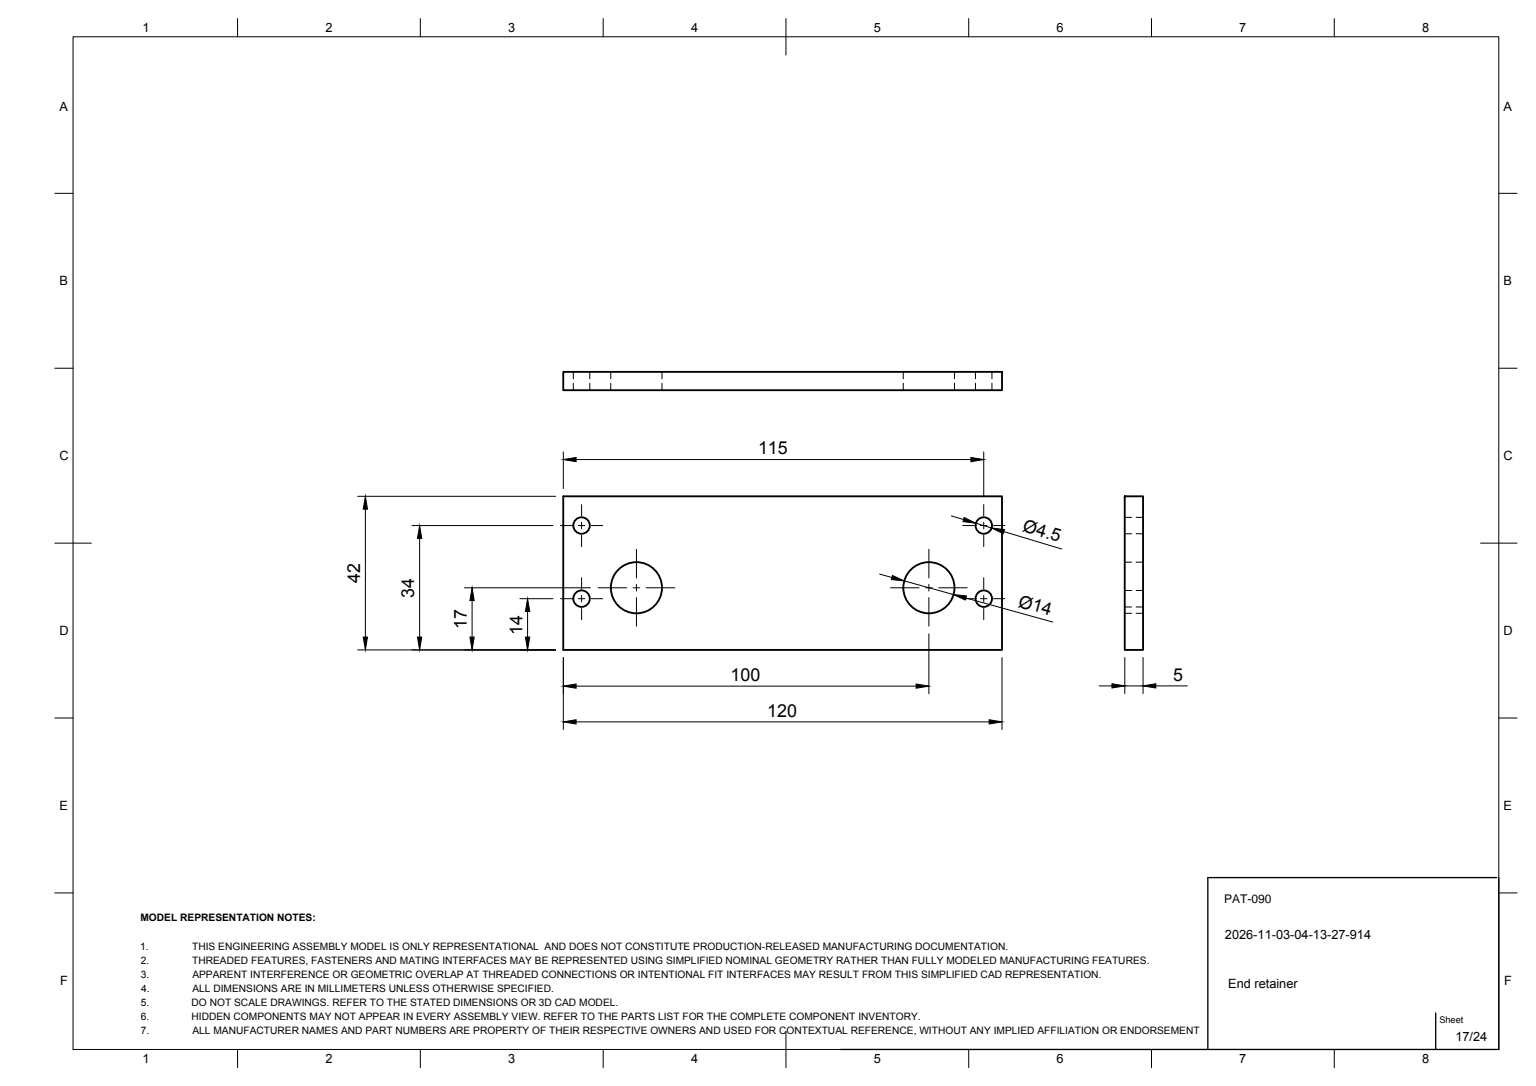
ISO-10303-21;
HEADER;
/* Generated by software containing ST-Developer
 * from STEP Tools, Inc. (www.steptools.com) 
 */

FILE_DESCRIPTION(
/* description */ ('Round-Shaft Linear Stage with Ball Bushings'),
/* implementation_level */ '2;1');

FILE_NAME(
/* name */ 'End retainer.step',
/* time_stamp */ '2026-10-27T10:47:55-07:00',
/* author */ (''),
/* organization */ (''),
/* preprocessor_version */ 'ST-DEVELOPER v20.2',
/* originating_system */ 'Autodesk Translation Framework v15.17.0.0',
/* authorisation */ '');

FILE_SCHEMA (('AUTOMOTIVE_DESIGN { 1 0 10303 214 3 1 1 }'));
ENDSEC;

DATA;
#10=MECHANICAL_DESIGN_GEOMETRIC_PRESENTATION_REPRESENTATION('',(#313),#7835);
#271=SHAPE_REPRESENTATION_RELATIONSHIP('SRR','None',#7960,#292);
#292=ADVANCED_BREP_SHAPE_REPRESENTATION('',(#333),#7824);
#313=STYLED_ITEM('',(#8130),#333);
#333=MANIFOLD_SOLID_BREP('Body1',#4404);
#407=FACE_BOUND('',#1086,.T.);
#408=FACE_BOUND('',#1087,.T.);
#409=FACE_BOUND('',#1088,.T.);
#410=FACE_BOUND('',#1089,.T.);
#411=FACE_BOUND('',#1090,.T.);
#412=FACE_BOUND('',#1091,.T.);
#413=FACE_BOUND('',#1094,.T.);
#414=FACE_BOUND('',#1095,.T.);
#415=FACE_BOUND('',#1096,.T.);
#416=FACE_BOUND('',#1097,.T.);
#417=FACE_BOUND('',#1098,.T.);
#418=FACE_BOUND('',#1099,.T.);
#544=PLANE('',#4921);
#545=PLANE('',#4922);
#546=PLANE('',#4923);
#547=PLANE('',#4924);
#548=PLANE('',#4925);
#549=PLANE('',#4926);
#754=FACE_OUTER_BOUND('',#1078,.T.);
#755=FACE_OUTER_BOUND('',#1079,.T.);
#756=FACE_OUTER_BOUND('',#1080,.T.);
#757=FACE_OUTER_BOUND('',#1081,.T.);
#758=FACE_OUTER_BOUND('',#1082,.T.);
#759=FACE_OUTER_BOUND('',#1083,.T.);
#760=FACE_OUTER_BOUND('',#1084,.T.);
#761=FACE_OUTER_BOUND('',#1085,.T.);
#762=FACE_OUTER_BOUND('',#1092,.T.);
#763=FACE_OUTER_BOUND('',#1093,.T.);
#764=FACE_OUTER_BOUND('',#1100,.T.);
#765=FACE_OUTER_BOUND('',#1101,.T.);
#1078=EDGE_LOOP('',(#3566,#3567,#3568,#3569));
#1079=EDGE_LOOP('',(#3570,#3571,#3572,#3573));
#1080=EDGE_LOOP('',(#3574,#3575,#3576,#3577));
#1081=EDGE_LOOP('',(#3578,#3579,#3580,#3581));
#1082=EDGE_LOOP('',(#3582,#3583,#3584,#3585));
#1083=EDGE_LOOP('',(#3586,#3587,#3588,#3589));
#1084=EDGE_LOOP('',(#3590,#3591,#3592,#3593));
#1085=EDGE_LOOP('',(#3594,#3595,#3596,#3597));
#1086=EDGE_LOOP('',(#3598));
#1087=EDGE_LOOP('',(#3599));
#1088=EDGE_LOOP('',(#3600));
#1089=EDGE_LOOP('',(#3601));
#1090=EDGE_LOOP('',(#3602));
#1091=EDGE_LOOP('',(#3603));
#1092=EDGE_LOOP('',(#3604,#3605,#3606,#3607));
#1093=EDGE_LOOP('',(#3608,#3609,#3610,#3611));
#1094=EDGE_LOOP('',(#3612));
#1095=EDGE_LOOP('',(#3613));
#1096=EDGE_LOOP('',(#3614));
#1097=EDGE_LOOP('',(#3615));
#1098=EDGE_LOOP('',(#3616));
#1099=EDGE_LOOP('',(#3617));
#1100=EDGE_LOOP('',(#3618,#3619,#3620,#3621));
#1101=EDGE_LOOP('',(#3622,#3623,#3624,#3625));
#1434=LINE('',#7202,#1774);
#1435=LINE('',#7208,#1775);
#1436=LINE('',#7214,#1776);
#1437=LINE('',#7220,#1777);
#1438=LINE('',#7226,#1778);
#1439=LINE('',#7232,#1779);
#1440=LINE('',#7237,#1780);
#1441=LINE('',#7239,#1781);
#1442=LINE('',#7241,#1782);
#1443=LINE('',#7242,#1783);
#1444=LINE('',#7245,#1784);
#1445=LINE('',#7247,#1785);
#1446=LINE('',#7248,#1786);
#1447=LINE('',#7251,#1787);
#1448=LINE('',#7253,#1788);
#1449=LINE('',#7254,#1789);
#1450=LINE('',#7256,#1790);
#1451=LINE('',#7257,#1791);
#1774=VECTOR('',#5873,0.225);
#1775=VECTOR('',#5880,0.225);
#1776=VECTOR('',#5887,0.225);
#1777=VECTOR('',#5894,0.225);
#1778=VECTOR('',#5901,0.7);
#1779=VECTOR('',#5908,0.7);
#1780=VECTOR('',#5913,1.);
#1781=VECTOR('',#5914,1.);
#1782=VECTOR('',#5915,1.);
#1783=VECTOR('',#5916,1.);
#1784=VECTOR('',#5919,1.);
#1785=VECTOR('',#5920,1.);
#1786=VECTOR('',#5921,1.);
#1787=VECTOR('',#5924,1.);
#1788=VECTOR('',#5925,1.);
#1789=VECTOR('',#5926,1.);
#1790=VECTOR('',#5929,1.);
#1791=VECTOR('',#5930,1.);
#2030=CIRCLE('',#4904,0.225);
#2031=CIRCLE('',#4905,0.225);
#2032=CIRCLE('',#4907,0.225);
#2033=CIRCLE('',#4908,0.225);
#2034=CIRCLE('',#4910,0.225);
#2035=CIRCLE('',#4911,0.225);
#2036=CIRCLE('',#4913,0.225);
#2037=CIRCLE('',#4914,0.225);
#2038=CIRCLE('',#4916,0.7);
#2039=CIRCLE('',#4917,0.7);
#2040=CIRCLE('',#4919,0.7);
#2041=CIRCLE('',#4920,0.7);
#2307=VERTEX_POINT('',#7199);
#2308=VERTEX_POINT('',#7201);
#2309=VERTEX_POINT('',#7205);
#2310=VERTEX_POINT('',#7207);
#2311=VERTEX_POINT('',#7211);
#2312=VERTEX_POINT('',#7213);
#2313=VERTEX_POINT('',#7217);
#2314=VERTEX_POINT('',#7219);
#2315=VERTEX_POINT('',#7223);
#2316=VERTEX_POINT('',#7225);
#2317=VERTEX_POINT('',#7229);
#2318=VERTEX_POINT('',#7231);
#2319=VERTEX_POINT('',#7235);
#2320=VERTEX_POINT('',#7236);
#2321=VERTEX_POINT('',#7238);
#2322=VERTEX_POINT('',#7240);
#2323=VERTEX_POINT('',#7244);
#2324=VERTEX_POINT('',#7246);
#2325=VERTEX_POINT('',#7250);
#2326=VERTEX_POINT('',#7252);
#2751=EDGE_CURVE('',#2307,#2307,#2030,.T.);
#2752=EDGE_CURVE('',#2307,#2308,#1434,.T.);
#2753=EDGE_CURVE('',#2308,#2308,#2031,.T.);
#2754=EDGE_CURVE('',#2309,#2309,#2032,.T.);
#2755=EDGE_CURVE('',#2309,#2310,#1435,.T.);
#2756=EDGE_CURVE('',#2310,#2310,#2033,.T.);
#2757=EDGE_CURVE('',#2311,#2311,#2034,.T.);
#2758=EDGE_CURVE('',#2311,#2312,#1436,.T.);
#2759=EDGE_CURVE('',#2312,#2312,#2035,.T.);
#2760=EDGE_CURVE('',#2313,#2313,#2036,.T.);
#2761=EDGE_CURVE('',#2313,#2314,#1437,.T.);
#2762=EDGE_CURVE('',#2314,#2314,#2037,.T.);
#2763=EDGE_CURVE('',#2315,#2315,#2038,.T.);
#2764=EDGE_CURVE('',#2315,#2316,#1438,.T.);
#2765=EDGE_CURVE('',#2316,#2316,#2039,.T.);
#2766=EDGE_CURVE('',#2317,#2317,#2040,.T.);
#2767=EDGE_CURVE('',#2317,#2318,#1439,.T.);
#2768=EDGE_CURVE('',#2318,#2318,#2041,.T.);
#2769=EDGE_CURVE('',#2319,#2320,#1440,.T.);
#2770=EDGE_CURVE('',#2320,#2321,#1441,.T.);
#2771=EDGE_CURVE('',#2322,#2321,#1442,.T.);
#2772=EDGE_CURVE('',#2319,#2322,#1443,.T.);
#2773=EDGE_CURVE('',#2323,#2319,#1444,.T.);
#2774=EDGE_CURVE('',#2324,#2322,#1445,.T.);
#2775=EDGE_CURVE('',#2323,#2324,#1446,.T.);
#2776=EDGE_CURVE('',#2325,#2323,#1447,.T.);
#2777=EDGE_CURVE('',#2326,#2324,#1448,.T.);
#2778=EDGE_CURVE('',#2325,#2326,#1449,.T.);
#2779=EDGE_CURVE('',#2320,#2325,#1450,.T.);
#2780=EDGE_CURVE('',#2321,#2326,#1451,.T.);
#3566=ORIENTED_EDGE('',*,*,#2751,.F.);
#3567=ORIENTED_EDGE('',*,*,#2752,.T.);
#3568=ORIENTED_EDGE('',*,*,#2753,.F.);
#3569=ORIENTED_EDGE('',*,*,#2752,.F.);
#3570=ORIENTED_EDGE('',*,*,#2754,.F.);
#3571=ORIENTED_EDGE('',*,*,#2755,.T.);
#3572=ORIENTED_EDGE('',*,*,#2756,.F.);
#3573=ORIENTED_EDGE('',*,*,#2755,.F.);
#3574=ORIENTED_EDGE('',*,*,#2757,.F.);
#3575=ORIENTED_EDGE('',*,*,#2758,.T.);
#3576=ORIENTED_EDGE('',*,*,#2759,.F.);
#3577=ORIENTED_EDGE('',*,*,#2758,.F.);
#3578=ORIENTED_EDGE('',*,*,#2760,.F.);
#3579=ORIENTED_EDGE('',*,*,#2761,.T.);
#3580=ORIENTED_EDGE('',*,*,#2762,.F.);
#3581=ORIENTED_EDGE('',*,*,#2761,.F.);
#3582=ORIENTED_EDGE('',*,*,#2763,.F.);
#3583=ORIENTED_EDGE('',*,*,#2764,.T.);
#3584=ORIENTED_EDGE('',*,*,#2765,.F.);
#3585=ORIENTED_EDGE('',*,*,#2764,.F.);
#3586=ORIENTED_EDGE('',*,*,#2766,.F.);
#3587=ORIENTED_EDGE('',*,*,#2767,.T.);
#3588=ORIENTED_EDGE('',*,*,#2768,.F.);
#3589=ORIENTED_EDGE('',*,*,#2767,.F.);
#3590=ORIENTED_EDGE('',*,*,#2769,.T.);
#3591=ORIENTED_EDGE('',*,*,#2770,.T.);
#3592=ORIENTED_EDGE('',*,*,#2771,.F.);
#3593=ORIENTED_EDGE('',*,*,#2772,.F.);
#3594=ORIENTED_EDGE('',*,*,#2773,.T.);
#3595=ORIENTED_EDGE('',*,*,#2772,.T.);
#3596=ORIENTED_EDGE('',*,*,#2774,.F.);
#3597=ORIENTED_EDGE('',*,*,#2775,.F.);
#3598=ORIENTED_EDGE('',*,*,#2768,.T.);
#3599=ORIENTED_EDGE('',*,*,#2765,.T.);
#3600=ORIENTED_EDGE('',*,*,#2762,.T.);
#3601=ORIENTED_EDGE('',*,*,#2759,.T.);
#3602=ORIENTED_EDGE('',*,*,#2756,.T.);
#3603=ORIENTED_EDGE('',*,*,#2753,.T.);
#3604=ORIENTED_EDGE('',*,*,#2776,.T.);
#3605=ORIENTED_EDGE('',*,*,#2775,.T.);
#3606=ORIENTED_EDGE('',*,*,#2777,.F.);
#3607=ORIENTED_EDGE('',*,*,#2778,.F.);
#3608=ORIENTED_EDGE('',*,*,#2779,.T.);
#3609=ORIENTED_EDGE('',*,*,#2778,.T.);
#3610=ORIENTED_EDGE('',*,*,#2780,.F.);
#3611=ORIENTED_EDGE('',*,*,#2770,.F.);
#3612=ORIENTED_EDGE('',*,*,#2766,.T.);
#3613=ORIENTED_EDGE('',*,*,#2763,.T.);
#3614=ORIENTED_EDGE('',*,*,#2760,.T.);
#3615=ORIENTED_EDGE('',*,*,#2757,.T.);
#3616=ORIENTED_EDGE('',*,*,#2754,.T.);
#3617=ORIENTED_EDGE('',*,*,#2751,.T.);
#3618=ORIENTED_EDGE('',*,*,#2780,.T.);
#3619=ORIENTED_EDGE('',*,*,#2777,.T.);
#3620=ORIENTED_EDGE('',*,*,#2774,.T.);
#3621=ORIENTED_EDGE('',*,*,#2771,.T.);
#3622=ORIENTED_EDGE('',*,*,#2779,.F.);
#3623=ORIENTED_EDGE('',*,*,#2769,.F.);
#3624=ORIENTED_EDGE('',*,*,#2773,.F.);
#3625=ORIENTED_EDGE('',*,*,#2776,.F.);
#4100=CYLINDRICAL_SURFACE('',#4903,0.225);
#4101=CYLINDRICAL_SURFACE('',#4906,0.225);
#4102=CYLINDRICAL_SURFACE('',#4909,0.225);
#4103=CYLINDRICAL_SURFACE('',#4912,0.225);
#4104=CYLINDRICAL_SURFACE('',#4915,0.7);
#4105=CYLINDRICAL_SURFACE('',#4918,0.7);
#4273=ADVANCED_FACE('',(#754),#4100,.F.);
#4274=ADVANCED_FACE('',(#755),#4101,.F.);
#4275=ADVANCED_FACE('',(#756),#4102,.F.);
#4276=ADVANCED_FACE('',(#757),#4103,.F.);
#4277=ADVANCED_FACE('',(#758),#4104,.F.);
#4278=ADVANCED_FACE('',(#759),#4105,.F.);
#4279=ADVANCED_FACE('',(#760),#544,.T.);
#4280=ADVANCED_FACE('',(#761,#407,#408,#409,#410,#411,#412),#545,.T.);
#4281=ADVANCED_FACE('',(#762),#546,.T.);
#4282=ADVANCED_FACE('',(#763,#413,#414,#415,#416,#417,#418),#547,.T.);
#4283=ADVANCED_FACE('',(#764),#548,.T.);
#4284=ADVANCED_FACE('',(#765),#549,.F.);
#4404=CLOSED_SHELL('',(#4273,#4274,#4275,#4276,#4277,#4278,#4279,#4280,
#4281,#4282,#4283,#4284));
#4902=AXIS2_PLACEMENT_3D('',#7197,#5867,#5868);
#4903=AXIS2_PLACEMENT_3D('',#7198,#5869,#5870);
#4904=AXIS2_PLACEMENT_3D('',#7200,#5871,#5872);
#4905=AXIS2_PLACEMENT_3D('',#7203,#5874,#5875);
#4906=AXIS2_PLACEMENT_3D('',#7204,#5876,#5877);
#4907=AXIS2_PLACEMENT_3D('',#7206,#5878,#5879);
#4908=AXIS2_PLACEMENT_3D('',#7209,#5881,#5882);
#4909=AXIS2_PLACEMENT_3D('',#7210,#5883,#5884);
#4910=AXIS2_PLACEMENT_3D('',#7212,#5885,#5886);
#4911=AXIS2_PLACEMENT_3D('',#7215,#5888,#5889);
#4912=AXIS2_PLACEMENT_3D('',#7216,#5890,#5891);
#4913=AXIS2_PLACEMENT_3D('',#7218,#5892,#5893);
#4914=AXIS2_PLACEMENT_3D('',#7221,#5895,#5896);
#4915=AXIS2_PLACEMENT_3D('',#7222,#5897,#5898);
#4916=AXIS2_PLACEMENT_3D('',#7224,#5899,#5900);
#4917=AXIS2_PLACEMENT_3D('',#7227,#5902,#5903);
#4918=AXIS2_PLACEMENT_3D('',#7228,#5904,#5905);
#4919=AXIS2_PLACEMENT_3D('',#7230,#5906,#5907);
#4920=AXIS2_PLACEMENT_3D('',#7233,#5909,#5910);
#4921=AXIS2_PLACEMENT_3D('',#7234,#5911,#5912);
#4922=AXIS2_PLACEMENT_3D('',#7243,#5917,#5918);
#4923=AXIS2_PLACEMENT_3D('',#7249,#5922,#5923);
#4924=AXIS2_PLACEMENT_3D('',#7255,#5927,#5928);
#4925=AXIS2_PLACEMENT_3D('',#7258,#5931,#5932);
#4926=AXIS2_PLACEMENT_3D('',#7259,#5933,#5934);
#5867=DIRECTION('axis',(0.,0.,1.));
#5868=DIRECTION('refdir',(1.,0.,0.));
#5869=DIRECTION('center_axis',(1.,0.,0.));
#5870=DIRECTION('ref_axis',(0.,0.,-1.));
#5871=DIRECTION('center_axis',(1.,0.,0.));
#5872=DIRECTION('ref_axis',(0.,0.,-1.));
#5873=DIRECTION('',(1.,0.,0.));
#5874=DIRECTION('center_axis',(-1.,0.,0.));
#5875=DIRECTION('ref_axis',(0.,0.,-1.));
#5876=DIRECTION('center_axis',(1.,0.,0.));
#5877=DIRECTION('ref_axis',(0.,0.,-1.));
#5878=DIRECTION('center_axis',(1.,0.,0.));
#5879=DIRECTION('ref_axis',(0.,0.,-1.));
#5880=DIRECTION('',(1.,0.,0.));
#5881=DIRECTION('center_axis',(-1.,0.,0.));
#5882=DIRECTION('ref_axis',(0.,0.,-1.));
#5883=DIRECTION('center_axis',(1.,0.,0.));
#5884=DIRECTION('ref_axis',(0.,0.,-1.));
#5885=DIRECTION('center_axis',(1.,0.,0.));
#5886=DIRECTION('ref_axis',(0.,0.,-1.));
#5887=DIRECTION('',(1.,0.,0.));
#5888=DIRECTION('center_axis',(-1.,0.,0.));
#5889=DIRECTION('ref_axis',(0.,0.,-1.));
#5890=DIRECTION('center_axis',(1.,0.,0.));
#5891=DIRECTION('ref_axis',(0.,0.,-1.));
#5892=DIRECTION('center_axis',(1.,0.,0.));
#5893=DIRECTION('ref_axis',(0.,0.,-1.));
#5894=DIRECTION('',(1.,0.,0.));
#5895=DIRECTION('center_axis',(-1.,0.,0.));
#5896=DIRECTION('ref_axis',(0.,0.,-1.));
#5897=DIRECTION('center_axis',(1.,0.,0.));
#5898=DIRECTION('ref_axis',(0.,0.,-1.));
#5899=DIRECTION('center_axis',(1.,0.,0.));
#5900=DIRECTION('ref_axis',(0.,0.,-1.));
#5901=DIRECTION('',(1.,0.,0.));
#5902=DIRECTION('center_axis',(-1.,0.,0.));
#5903=DIRECTION('ref_axis',(0.,0.,-1.));
#5904=DIRECTION('center_axis',(1.,0.,0.));
#5905=DIRECTION('ref_axis',(0.,0.,-1.));
#5906=DIRECTION('center_axis',(1.,0.,0.));
#5907=DIRECTION('ref_axis',(0.,0.,-1.));
#5908=DIRECTION('',(1.,0.,0.));
#5909=DIRECTION('center_axis',(-1.,0.,0.));
#5910=DIRECTION('ref_axis',(0.,0.,-1.));
#5911=DIRECTION('center_axis',(0.,1.,0.));
#5912=DIRECTION('ref_axis',(-1.,0.,0.));
#5913=DIRECTION('',(-1.,0.,0.));
#5914=DIRECTION('',(0.,0.,1.));
#5915=DIRECTION('',(-1.,0.,0.));
#5916=DIRECTION('',(0.,0.,1.));
#5917=DIRECTION('center_axis',(1.,0.,0.));
#5918=DIRECTION('ref_axis',(0.,1.,0.));
#5919=DIRECTION('',(0.,1.,0.));
#5920=DIRECTION('',(0.,1.,0.));
#5921=DIRECTION('',(0.,0.,1.));
#5922=DIRECTION('center_axis',(0.,-1.,0.));
#5923=DIRECTION('ref_axis',(1.,0.,0.));
#5924=DIRECTION('',(1.,0.,0.));
#5925=DIRECTION('',(1.,0.,0.));
#5926=DIRECTION('',(0.,0.,1.));
#5927=DIRECTION('center_axis',(-1.,0.,0.));
#5928=DIRECTION('ref_axis',(0.,-1.,0.));
#5929=DIRECTION('',(0.,-1.,0.));
#5930=DIRECTION('',(0.,-1.,0.));
#5931=DIRECTION('center_axis',(0.,0.,1.));
#5932=DIRECTION('ref_axis',(1.,0.,0.));
#5933=DIRECTION('center_axis',(0.,0.,1.));
#5934=DIRECTION('ref_axis',(1.,0.,0.));
#7197=CARTESIAN_POINT('',(0.,0.,0.));
#7198=CARTESIAN_POINT('Origin',(9.9,5.5,3.));
#7199=CARTESIAN_POINT('',(10.,5.5,3.225));
#7200=CARTESIAN_POINT('Origin',(10.,5.5,3.));
#7201=CARTESIAN_POINT('',(10.5,5.5,3.225));
#7202=CARTESIAN_POINT('',(9.9,5.5,3.225));
#7203=CARTESIAN_POINT('Origin',(10.5,5.5,3.));
#7204=CARTESIAN_POINT('Origin',(9.9,-5.5,5.));
#7205=CARTESIAN_POINT('',(10.,-5.5,5.225));
#7206=CARTESIAN_POINT('Origin',(10.,-5.5,5.));
#7207=CARTESIAN_POINT('',(10.5,-5.5,5.225));
#7208=CARTESIAN_POINT('',(9.9,-5.5,5.225));
#7209=CARTESIAN_POINT('Origin',(10.5,-5.5,5.));
#7210=CARTESIAN_POINT('Origin',(9.9,-5.5,3.));
#7211=CARTESIAN_POINT('',(10.,-5.5,3.225));
#7212=CARTESIAN_POINT('Origin',(10.,-5.5,3.));
#7213=CARTESIAN_POINT('',(10.5,-5.5,3.225));
#7214=CARTESIAN_POINT('',(9.9,-5.5,3.225));
#7215=CARTESIAN_POINT('Origin',(10.5,-5.5,3.));
#7216=CARTESIAN_POINT('Origin',(9.9,5.5,5.));
#7217=CARTESIAN_POINT('',(10.,5.5,5.225));
#7218=CARTESIAN_POINT('Origin',(10.,5.5,5.));
#7219=CARTESIAN_POINT('',(10.5,5.5,5.225));
#7220=CARTESIAN_POINT('',(9.9,5.5,5.225));
#7221=CARTESIAN_POINT('Origin',(10.5,5.5,5.));
#7222=CARTESIAN_POINT('Origin',(9.9,-4.,3.3));
#7223=CARTESIAN_POINT('',(10.,-4.,4.));
#7224=CARTESIAN_POINT('Origin',(10.,-4.,3.3));
#7225=CARTESIAN_POINT('',(10.5,-4.,4.));
#7226=CARTESIAN_POINT('',(9.9,-4.,4.));
#7227=CARTESIAN_POINT('Origin',(10.5,-4.,3.3));
#7228=CARTESIAN_POINT('Origin',(9.9,4.,3.3));
#7229=CARTESIAN_POINT('',(10.,4.,4.));
#7230=CARTESIAN_POINT('Origin',(10.,4.,3.3));
#7231=CARTESIAN_POINT('',(10.5,4.,4.));
#7232=CARTESIAN_POINT('',(9.9,4.,4.));
#7233=CARTESIAN_POINT('Origin',(10.5,4.,3.3));
#7234=CARTESIAN_POINT('Origin',(10.5,6.,1.6));
#7235=CARTESIAN_POINT('',(10.5,6.,1.6));
#7236=CARTESIAN_POINT('',(10.,6.,1.6));
#7237=CARTESIAN_POINT('',(10.5,6.,1.6));
#7238=CARTESIAN_POINT('',(10.,6.,5.8));
#7239=CARTESIAN_POINT('',(10.,6.,1.6));
#7240=CARTESIAN_POINT('',(10.5,6.,5.8));
#7241=CARTESIAN_POINT('',(10.5,6.,5.8));
#7242=CARTESIAN_POINT('',(10.5,6.,1.6));
#7243=CARTESIAN_POINT('Origin',(10.5,-6.,1.6));
#7244=CARTESIAN_POINT('',(10.5,-6.,1.6));
#7245=CARTESIAN_POINT('',(10.5,-6.,1.6));
#7246=CARTESIAN_POINT('',(10.5,-6.,5.8));
#7247=CARTESIAN_POINT('',(10.5,-6.,5.8));
#7248=CARTESIAN_POINT('',(10.5,-6.,1.6));
#7249=CARTESIAN_POINT('Origin',(10.,-6.,1.6));
#7250=CARTESIAN_POINT('',(10.,-6.,1.6));
#7251=CARTESIAN_POINT('',(10.,-6.,1.6));
#7252=CARTESIAN_POINT('',(10.,-6.,5.8));
#7253=CARTESIAN_POINT('',(10.,-6.,5.8));
#7254=CARTESIAN_POINT('',(10.,-6.,1.6));
#7255=CARTESIAN_POINT('Origin',(10.,6.,1.6));
#7256=CARTESIAN_POINT('',(10.,6.,1.6));
#7257=CARTESIAN_POINT('',(10.,6.,5.8));
#7258=CARTESIAN_POINT('Origin',(10.25,0.,5.8));
#7259=CARTESIAN_POINT('Origin',(10.25,0.,1.6));
#7798=UNCERTAINTY_MEASURE_WITH_UNIT(LENGTH_MEASURE(0.001),#7836,
'DISTANCE_ACCURACY_VALUE',
'Maximum model space distance between geometric entities at asserted c
onnectivities');
#7809=UNCERTAINTY_MEASURE_WITH_UNIT(LENGTH_MEASURE(0.001),#7836,
'DISTANCE_ACCURACY_VALUE',
'Maximum model space distance between geometric entities at asserted c
onnectivities');
#7824=(
GEOMETRIC_REPRESENTATION_CONTEXT(3)
GLOBAL_UNCERTAINTY_ASSIGNED_CONTEXT((#7798))
GLOBAL_UNIT_ASSIGNED_CONTEXT((#7836,#7838,#7839))
REPRESENTATION_CONTEXT('','3D')
);
#7835=(
GEOMETRIC_REPRESENTATION_CONTEXT(3)
GLOBAL_UNCERTAINTY_ASSIGNED_CONTEXT((#7809))
GLOBAL_UNIT_ASSIGNED_CONTEXT((#7836,#7838,#7839))
REPRESENTATION_CONTEXT('','3D')
);
#7836=(
LENGTH_UNIT()
NAMED_UNIT(*)
SI_UNIT(.CENTI.,.METRE.)
);
#7838=(
NAMED_UNIT(*)
PLANE_ANGLE_UNIT()
SI_UNIT($,.RADIAN.)
);
#7839=(
NAMED_UNIT(*)
SI_UNIT($,.STERADIAN.)
SOLID_ANGLE_UNIT()
);
#7854=SHAPE_DEFINITION_REPRESENTATION(#7879,#7960);
#7879=PRODUCT_DEFINITION_SHAPE('',$,#7986);
#7960=SHAPE_REPRESENTATION('',(#4902),#7824);
#7971=PRODUCT_DEFINITION_CONTEXT('part definition',#8048,'design');
#7986=PRODUCT_DEFINITION('End retainer','End retainer',#8011,#7971);
#8011=PRODUCT_DEFINITION_FORMATION('',$,#8064);
#8048=APPLICATION_CONTEXT(
'Core Data for Automotive Mechanical Design Process');
#8049=PRODUCT_CONTEXT('part definition',#8048,'mechanical');
#8064=PRODUCT('End retainer','End retainer','End retainer',(#8049));
#8124=COLOUR_RGB('Light Blue',0.38,0.62,0.78);
#8125=FILL_AREA_STYLE_COLOUR('',#8124);
#8126=FILL_AREA_STYLE('',(#8125));
#8127=SURFACE_STYLE_FILL_AREA(#8126);
#8128=SURFACE_SIDE_STYLE('',(#8127));
#8129=SURFACE_STYLE_USAGE(.BOTH.,#8128);
#8130=PRESENTATION_STYLE_ASSIGNMENT((#8129));
ENDSEC;
END-ISO-10303-21;
